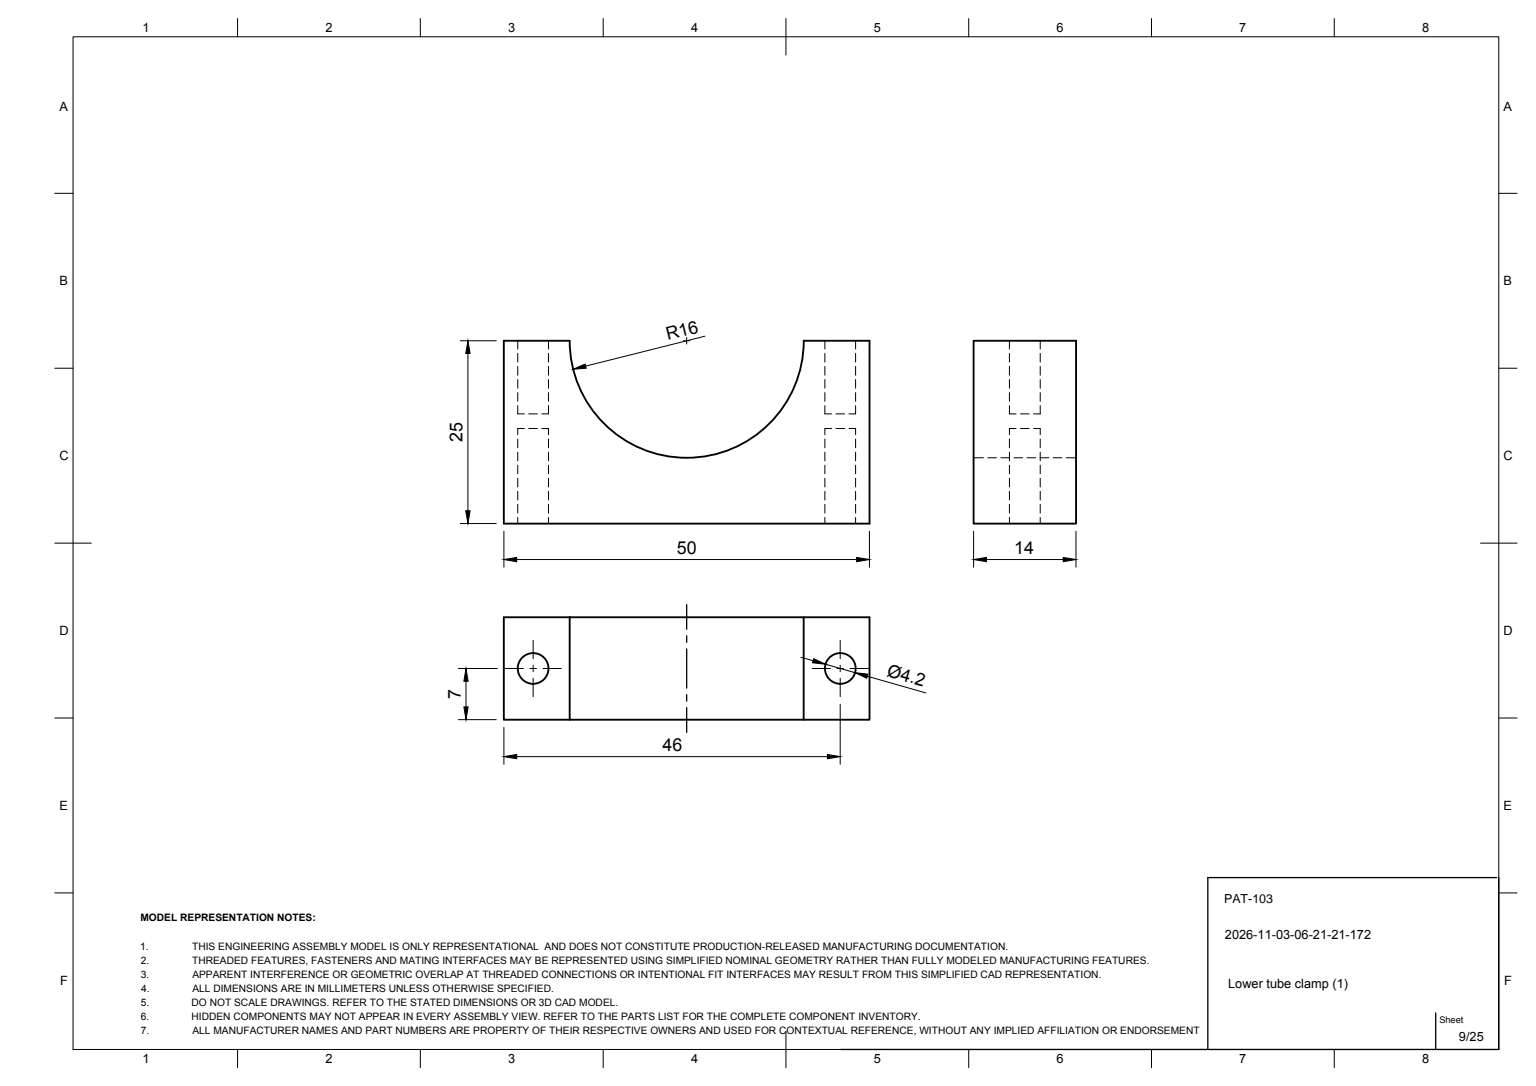
ISO-10303-21;
HEADER;
/* Generated by software containing ST-Developer
 * from STEP Tools, Inc. (www.steptools.com) 
 */

FILE_DESCRIPTION(
/* description */ ('Telescoping shaft support with lock collar'),
/* implementation_level */ '2;1');

FILE_NAME(
/* name */ 'Lower tube clamp (1).step',
/* time_stamp */ '2026-10-27T10:48:51-07:00',
/* author */ (''),
/* organization */ (''),
/* preprocessor_version */ 'ST-DEVELOPER v20.2',
/* originating_system */ 'Autodesk Translation Framework v15.17.0.0',
/* authorisation */ '');

FILE_SCHEMA (('AUTOMOTIVE_DESIGN { 1 0 10303 214 3 1 1 }'));
ENDSEC;

DATA;
#10=MECHANICAL_DESIGN_GEOMETRIC_PRESENTATION_REPRESENTATION('',(#245),#7349);
#205=SHAPE_REPRESENTATION_RELATIONSHIP('SRR','None',#7447,#225);
#225=ADVANCED_BREP_SHAPE_REPRESENTATION('',(#265),#7331);
#245=STYLED_ITEM('',(#7613),#265);
#265=MANIFOLD_SOLID_BREP('Body1',#3968);
#305=FACE_BOUND('',#818,.T.);
#306=FACE_BOUND('',#823,.T.);
#307=FACE_BOUND('',#825,.T.);
#308=FACE_BOUND('',#826,.T.);
#395=PLANE('',#4349);
#396=PLANE('',#4353);
#397=PLANE('',#4357);
#398=PLANE('',#4361);
#399=PLANE('',#4365);
#400=PLANE('',#4366);
#401=PLANE('',#4367);
#402=PLANE('',#4368);
#403=PLANE('',#4369);
#404=PLANE('',#4370);
#405=PLANE('',#4371);
#555=FACE_OUTER_BOUND('',#807,.T.);
#556=FACE_OUTER_BOUND('',#808,.T.);
#557=FACE_OUTER_BOUND('',#809,.T.);
#558=FACE_OUTER_BOUND('',#810,.T.);
#559=FACE_OUTER_BOUND('',#811,.T.);
#560=FACE_OUTER_BOUND('',#812,.T.);
#561=FACE_OUTER_BOUND('',#813,.T.);
#562=FACE_OUTER_BOUND('',#814,.T.);
#563=FACE_OUTER_BOUND('',#815,.T.);
#564=FACE_OUTER_BOUND('',#816,.T.);
#565=FACE_OUTER_BOUND('',#817,.T.);
#566=FACE_OUTER_BOUND('',#819,.T.);
#567=FACE_OUTER_BOUND('',#820,.T.);
#568=FACE_OUTER_BOUND('',#821,.T.);
#569=FACE_OUTER_BOUND('',#822,.T.);
#570=FACE_OUTER_BOUND('',#824,.T.);
#807=EDGE_LOOP('',(#2954,#2955,#2956,#2957));
#808=EDGE_LOOP('',(#2958));
#809=EDGE_LOOP('',(#2959,#2960,#2961,#2962));
#810=EDGE_LOOP('',(#2963));
#811=EDGE_LOOP('',(#2964,#2965,#2966,#2967));
#812=EDGE_LOOP('',(#2968));
#813=EDGE_LOOP('',(#2969,#2970,#2971,#2972));
#814=EDGE_LOOP('',(#2973));
#815=EDGE_LOOP('',(#2974,#2975,#2976,#2977));
#816=EDGE_LOOP('',(#2978,#2979,#2980,#2981,#2982,#2983));
#817=EDGE_LOOP('',(#2984,#2985,#2986,#2987));
#818=EDGE_LOOP('',(#2988));
#819=EDGE_LOOP('',(#2989,#2990,#2991,#2992));
#820=EDGE_LOOP('',(#2993,#2994,#2995,#2996));
#821=EDGE_LOOP('',(#2997,#2998,#2999,#3000,#3001,#3002));
#822=EDGE_LOOP('',(#3003,#3004,#3005,#3006));
#823=EDGE_LOOP('',(#3007));
#824=EDGE_LOOP('',(#3008,#3009,#3010,#3011));
#825=EDGE_LOOP('',(#3012));
#826=EDGE_LOOP('',(#3013));
#1111=LINE('',#6318,#1391);
#1112=LINE('',#6325,#1392);
#1113=LINE('',#6332,#1393);
#1114=LINE('',#6339,#1394);
#1115=LINE('',#6347,#1395);
#1116=LINE('',#6350,#1396);
#1117=LINE('',#6353,#1397);
#1118=LINE('',#6355,#1398);
#1119=LINE('',#6357,#1399);
#1120=LINE('',#6359,#1400);
#1121=LINE('',#6360,#1401);
#1122=LINE('',#6363,#1402);
#1123=LINE('',#6364,#1403);
#1124=LINE('',#6367,#1404);
#1125=LINE('',#6369,#1405);
#1126=LINE('',#6370,#1406);
#1127=LINE('',#6373,#1407);
#1128=LINE('',#6374,#1408);
#1129=LINE('',#6376,#1409);
#1130=LINE('',#6377,#1410);
#1391=VECTOR('',#5073,0.21);
#1392=VECTOR('',#5082,0.21);
#1393=VECTOR('',#5091,0.21);
#1394=VECTOR('',#5100,0.21);
#1395=VECTOR('',#5109,1.);
#1396=VECTOR('',#5112,1.);
#1397=VECTOR('',#5115,1.);
#1398=VECTOR('',#5116,1.);
#1399=VECTOR('',#5117,1.);
#1400=VECTOR('',#5118,1.);
#1401=VECTOR('',#5119,1.);
#1402=VECTOR('',#5122,1.);
#1403=VECTOR('',#5123,1.);
#1404=VECTOR('',#5126,1.);
#1405=VECTOR('',#5127,1.);
#1406=VECTOR('',#5128,1.);
#1407=VECTOR('',#5131,1.);
#1408=VECTOR('',#5132,1.);
#1409=VECTOR('',#5135,1.);
#1410=VECTOR('',#5136,1.);
#1659=CIRCLE('',#4347,0.21);
#1660=CIRCLE('',#4348,0.21);
#1661=CIRCLE('',#4351,0.21);
#1662=CIRCLE('',#4352,0.21);
#1663=CIRCLE('',#4355,0.21);
#1664=CIRCLE('',#4356,0.21);
#1665=CIRCLE('',#4359,0.21);
#1666=CIRCLE('',#4360,0.21);
#1667=CIRCLE('',#4363,1.6);
#1668=CIRCLE('',#4364,1.6);
#1902=VERTEX_POINT('',#6315);
#1903=VERTEX_POINT('',#6317);
#1904=VERTEX_POINT('',#6322);
#1905=VERTEX_POINT('',#6324);
#1906=VERTEX_POINT('',#6329);
#1907=VERTEX_POINT('',#6331);
#1908=VERTEX_POINT('',#6336);
#1909=VERTEX_POINT('',#6338);
#1910=VERTEX_POINT('',#6343);
#1911=VERTEX_POINT('',#6344);
#1912=VERTEX_POINT('',#6346);
#1913=VERTEX_POINT('',#6348);
#1914=VERTEX_POINT('',#6352);
#1915=VERTEX_POINT('',#6354);
#1916=VERTEX_POINT('',#6356);
#1917=VERTEX_POINT('',#6358);
#1918=VERTEX_POINT('',#6362);
#1919=VERTEX_POINT('',#6366);
#1920=VERTEX_POINT('',#6368);
#1921=VERTEX_POINT('',#6372);
#2289=EDGE_CURVE('',#1902,#1902,#1659,.T.);
#2290=EDGE_CURVE('',#1902,#1903,#1111,.T.);
#2291=EDGE_CURVE('',#1903,#1903,#1660,.T.);
#2292=EDGE_CURVE('',#1904,#1904,#1661,.T.);
#2293=EDGE_CURVE('',#1904,#1905,#1112,.T.);
#2294=EDGE_CURVE('',#1905,#1905,#1662,.T.);
#2295=EDGE_CURVE('',#1906,#1906,#1663,.T.);
#2296=EDGE_CURVE('',#1906,#1907,#1113,.T.);
#2297=EDGE_CURVE('',#1907,#1907,#1664,.T.);
#2298=EDGE_CURVE('',#1908,#1908,#1665,.T.);
#2299=EDGE_CURVE('',#1908,#1909,#1114,.T.);
#2300=EDGE_CURVE('',#1909,#1909,#1666,.T.);
#2301=EDGE_CURVE('',#1910,#1911,#1667,.T.);
#2302=EDGE_CURVE('',#1912,#1910,#1115,.T.);
#2303=EDGE_CURVE('',#1913,#1912,#1668,.T.);
#2304=EDGE_CURVE('',#1911,#1913,#1116,.T.);
#2305=EDGE_CURVE('',#1914,#1912,#1117,.T.);
#2306=EDGE_CURVE('',#1915,#1914,#1118,.T.);
#2307=EDGE_CURVE('',#1915,#1916,#1119,.T.);
#2308=EDGE_CURVE('',#1916,#1917,#1120,.T.);
#2309=EDGE_CURVE('',#1913,#1917,#1121,.T.);
#2310=EDGE_CURVE('',#1910,#1918,#1122,.T.);
#2311=EDGE_CURVE('',#1918,#1914,#1123,.T.);
#2312=EDGE_CURVE('',#1916,#1919,#1124,.T.);
#2313=EDGE_CURVE('',#1919,#1920,#1125,.T.);
#2314=EDGE_CURVE('',#1917,#1920,#1126,.T.);
#2315=EDGE_CURVE('',#1921,#1915,#1127,.T.);
#2316=EDGE_CURVE('',#1921,#1918,#1128,.T.);
#2317=EDGE_CURVE('',#1920,#1911,#1129,.T.);
#2318=EDGE_CURVE('',#1919,#1921,#1130,.T.);
#2954=ORIENTED_EDGE('',*,*,#2289,.F.);
#2955=ORIENTED_EDGE('',*,*,#2290,.T.);
#2956=ORIENTED_EDGE('',*,*,#2291,.F.);
#2957=ORIENTED_EDGE('',*,*,#2290,.F.);
#2958=ORIENTED_EDGE('',*,*,#2289,.T.);
#2959=ORIENTED_EDGE('',*,*,#2292,.F.);
#2960=ORIENTED_EDGE('',*,*,#2293,.T.);
#2961=ORIENTED_EDGE('',*,*,#2294,.F.);
#2962=ORIENTED_EDGE('',*,*,#2293,.F.);
#2963=ORIENTED_EDGE('',*,*,#2292,.T.);
#2964=ORIENTED_EDGE('',*,*,#2295,.F.);
#2965=ORIENTED_EDGE('',*,*,#2296,.T.);
#2966=ORIENTED_EDGE('',*,*,#2297,.T.);
#2967=ORIENTED_EDGE('',*,*,#2296,.F.);
#2968=ORIENTED_EDGE('',*,*,#2297,.F.);
#2969=ORIENTED_EDGE('',*,*,#2298,.F.);
#2970=ORIENTED_EDGE('',*,*,#2299,.T.);
#2971=ORIENTED_EDGE('',*,*,#2300,.T.);
#2972=ORIENTED_EDGE('',*,*,#2299,.F.);
#2973=ORIENTED_EDGE('',*,*,#2300,.F.);
#2974=ORIENTED_EDGE('',*,*,#2301,.F.);
#2975=ORIENTED_EDGE('',*,*,#2302,.F.);
#2976=ORIENTED_EDGE('',*,*,#2303,.F.);
#2977=ORIENTED_EDGE('',*,*,#2304,.F.);
#2978=ORIENTED_EDGE('',*,*,#2303,.T.);
#2979=ORIENTED_EDGE('',*,*,#2305,.F.);
#2980=ORIENTED_EDGE('',*,*,#2306,.F.);
#2981=ORIENTED_EDGE('',*,*,#2307,.T.);
#2982=ORIENTED_EDGE('',*,*,#2308,.T.);
#2983=ORIENTED_EDGE('',*,*,#2309,.F.);
#2984=ORIENTED_EDGE('',*,*,#2302,.T.);
#2985=ORIENTED_EDGE('',*,*,#2310,.T.);
#2986=ORIENTED_EDGE('',*,*,#2311,.T.);
#2987=ORIENTED_EDGE('',*,*,#2305,.T.);
#2988=ORIENTED_EDGE('',*,*,#2291,.T.);
#2989=ORIENTED_EDGE('',*,*,#2312,.T.);
#2990=ORIENTED_EDGE('',*,*,#2313,.T.);
#2991=ORIENTED_EDGE('',*,*,#2314,.F.);
#2992=ORIENTED_EDGE('',*,*,#2308,.F.);
#2993=ORIENTED_EDGE('',*,*,#2315,.T.);
#2994=ORIENTED_EDGE('',*,*,#2306,.T.);
#2995=ORIENTED_EDGE('',*,*,#2311,.F.);
#2996=ORIENTED_EDGE('',*,*,#2316,.F.);
#2997=ORIENTED_EDGE('',*,*,#2301,.T.);
#2998=ORIENTED_EDGE('',*,*,#2317,.F.);
#2999=ORIENTED_EDGE('',*,*,#2313,.F.);
#3000=ORIENTED_EDGE('',*,*,#2318,.T.);
#3001=ORIENTED_EDGE('',*,*,#2316,.T.);
#3002=ORIENTED_EDGE('',*,*,#2310,.F.);
#3003=ORIENTED_EDGE('',*,*,#2304,.T.);
#3004=ORIENTED_EDGE('',*,*,#2309,.T.);
#3005=ORIENTED_EDGE('',*,*,#2314,.T.);
#3006=ORIENTED_EDGE('',*,*,#2317,.T.);
#3007=ORIENTED_EDGE('',*,*,#2294,.T.);
#3008=ORIENTED_EDGE('',*,*,#2318,.F.);
#3009=ORIENTED_EDGE('',*,*,#2312,.F.);
#3010=ORIENTED_EDGE('',*,*,#2307,.F.);
#3011=ORIENTED_EDGE('',*,*,#2315,.F.);
#3012=ORIENTED_EDGE('',*,*,#2295,.T.);
#3013=ORIENTED_EDGE('',*,*,#2298,.T.);
#3684=CYLINDRICAL_SURFACE('',#4346,0.21);
#3685=CYLINDRICAL_SURFACE('',#4350,0.21);
#3686=CYLINDRICAL_SURFACE('',#4354,0.21);
#3687=CYLINDRICAL_SURFACE('',#4358,0.21);
#3688=CYLINDRICAL_SURFACE('',#4362,1.6);
#3798=ADVANCED_FACE('',(#555),#3684,.F.);
#3799=ADVANCED_FACE('',(#556),#395,.T.);
#3800=ADVANCED_FACE('',(#557),#3685,.F.);
#3801=ADVANCED_FACE('',(#558),#396,.T.);
#3802=ADVANCED_FACE('',(#559),#3686,.F.);
#3803=ADVANCED_FACE('',(#560),#397,.F.);
#3804=ADVANCED_FACE('',(#561),#3687,.F.);
#3805=ADVANCED_FACE('',(#562),#398,.F.);
#3806=ADVANCED_FACE('',(#563),#3688,.F.);
#3807=ADVANCED_FACE('',(#564),#399,.T.);
#3808=ADVANCED_FACE('',(#565,#305),#400,.T.);
#3809=ADVANCED_FACE('',(#566),#401,.T.);
#3810=ADVANCED_FACE('',(#567),#402,.T.);
#3811=ADVANCED_FACE('',(#568),#403,.T.);
#3812=ADVANCED_FACE('',(#569,#306),#404,.T.);
#3813=ADVANCED_FACE('',(#570,#307,#308),#405,.F.);
#3968=CLOSED_SHELL('',(#3798,#3799,#3800,#3801,#3802,#3803,#3804,#3805,
#3806,#3807,#3808,#3809,#3810,#3811,#3812,#3813));
#4345=AXIS2_PLACEMENT_3D('',#6313,#5067,#5068);
#4346=AXIS2_PLACEMENT_3D('',#6314,#5069,#5070);
#4347=AXIS2_PLACEMENT_3D('',#6316,#5071,#5072);
#4348=AXIS2_PLACEMENT_3D('',#6319,#5074,#5075);
#4349=AXIS2_PLACEMENT_3D('',#6320,#5076,#5077);
#4350=AXIS2_PLACEMENT_3D('',#6321,#5078,#5079);
#4351=AXIS2_PLACEMENT_3D('',#6323,#5080,#5081);
#4352=AXIS2_PLACEMENT_3D('',#6326,#5083,#5084);
#4353=AXIS2_PLACEMENT_3D('',#6327,#5085,#5086);
#4354=AXIS2_PLACEMENT_3D('',#6328,#5087,#5088);
#4355=AXIS2_PLACEMENT_3D('',#6330,#5089,#5090);
#4356=AXIS2_PLACEMENT_3D('',#6333,#5092,#5093);
#4357=AXIS2_PLACEMENT_3D('',#6334,#5094,#5095);
#4358=AXIS2_PLACEMENT_3D('',#6335,#5096,#5097);
#4359=AXIS2_PLACEMENT_3D('',#6337,#5098,#5099);
#4360=AXIS2_PLACEMENT_3D('',#6340,#5101,#5102);
#4361=AXIS2_PLACEMENT_3D('',#6341,#5103,#5104);
#4362=AXIS2_PLACEMENT_3D('',#6342,#5105,#5106);
#4363=AXIS2_PLACEMENT_3D('',#6345,#5107,#5108);
#4364=AXIS2_PLACEMENT_3D('',#6349,#5110,#5111);
#4365=AXIS2_PLACEMENT_3D('',#6351,#5113,#5114);
#4366=AXIS2_PLACEMENT_3D('',#6361,#5120,#5121);
#4367=AXIS2_PLACEMENT_3D('',#6365,#5124,#5125);
#4368=AXIS2_PLACEMENT_3D('',#6371,#5129,#5130);
#4369=AXIS2_PLACEMENT_3D('',#6375,#5133,#5134);
#4370=AXIS2_PLACEMENT_3D('',#6378,#5137,#5138);
#4371=AXIS2_PLACEMENT_3D('',#6379,#5139,#5140);
#5067=DIRECTION('axis',(0.,0.,1.));
#5068=DIRECTION('refdir',(1.,0.,0.));
#5069=DIRECTION('center_axis',(0.,0.,1.));
#5070=DIRECTION('ref_axis',(1.,0.,0.));
#5071=DIRECTION('center_axis',(0.,0.,1.));
#5072=DIRECTION('ref_axis',(1.,0.,0.));
#5073=DIRECTION('',(0.,0.,1.));
#5074=DIRECTION('center_axis',(0.,0.,-1.));
#5075=DIRECTION('ref_axis',(1.,0.,0.));
#5076=DIRECTION('center_axis',(0.,0.,1.));
#5077=DIRECTION('ref_axis',(1.,0.,0.));
#5078=DIRECTION('center_axis',(0.,0.,1.));
#5079=DIRECTION('ref_axis',(1.,0.,0.));
#5080=DIRECTION('center_axis',(0.,0.,1.));
#5081=DIRECTION('ref_axis',(1.,0.,0.));
#5082=DIRECTION('',(0.,0.,1.));
#5083=DIRECTION('center_axis',(0.,0.,-1.));
#5084=DIRECTION('ref_axis',(1.,0.,0.));
#5085=DIRECTION('center_axis',(0.,0.,1.));
#5086=DIRECTION('ref_axis',(1.,0.,0.));
#5087=DIRECTION('center_axis',(0.,0.,1.));
#5088=DIRECTION('ref_axis',(1.,0.,0.));
#5089=DIRECTION('center_axis',(0.,0.,1.));
#5090=DIRECTION('ref_axis',(1.,0.,0.));
#5091=DIRECTION('',(0.,0.,1.));
#5092=DIRECTION('center_axis',(0.,0.,1.));
#5093=DIRECTION('ref_axis',(1.,0.,0.));
#5094=DIRECTION('center_axis',(0.,0.,1.));
#5095=DIRECTION('ref_axis',(1.,0.,0.));
#5096=DIRECTION('center_axis',(0.,0.,1.));
#5097=DIRECTION('ref_axis',(1.,0.,0.));
#5098=DIRECTION('center_axis',(0.,0.,1.));
#5099=DIRECTION('ref_axis',(1.,0.,0.));
#5100=DIRECTION('',(0.,0.,1.));
#5101=DIRECTION('center_axis',(0.,0.,1.));
#5102=DIRECTION('ref_axis',(1.,0.,0.));
#5103=DIRECTION('center_axis',(0.,0.,1.));
#5104=DIRECTION('ref_axis',(1.,0.,0.));
#5105=DIRECTION('center_axis',(1.,0.,0.));
#5106=DIRECTION('ref_axis',(0.,0.,-1.));
#5107=DIRECTION('center_axis',(1.,0.,0.));
#5108=DIRECTION('ref_axis',(0.,0.,-1.));
#5109=DIRECTION('',(-1.,0.,0.));
#5110=DIRECTION('center_axis',(-1.,0.,0.));
#5111=DIRECTION('ref_axis',(0.,0.,-1.));
#5112=DIRECTION('',(1.,0.,0.));
#5113=DIRECTION('center_axis',(1.,0.,0.));
#5114=DIRECTION('ref_axis',(0.,1.,0.));
#5115=DIRECTION('',(0.,1.,0.));
#5116=DIRECTION('',(0.,0.,1.));
#5117=DIRECTION('',(0.,1.,0.));
#5118=DIRECTION('',(0.,0.,1.));
#5119=DIRECTION('',(0.,1.,0.));
#5120=DIRECTION('center_axis',(0.,0.,1.));
#5121=DIRECTION('ref_axis',(1.,0.,0.));
#5122=DIRECTION('',(0.,-1.,0.));
#5123=DIRECTION('',(1.,0.,0.));
#5124=DIRECTION('center_axis',(0.,1.,0.));
#5125=DIRECTION('ref_axis',(-1.,0.,0.));
#5126=DIRECTION('',(-1.,0.,0.));
#5127=DIRECTION('',(0.,0.,1.));
#5128=DIRECTION('',(-1.,0.,0.));
#5129=DIRECTION('center_axis',(0.,-1.,0.));
#5130=DIRECTION('ref_axis',(1.,0.,0.));
#5131=DIRECTION('',(1.,0.,0.));
#5132=DIRECTION('',(0.,0.,1.));
#5133=DIRECTION('center_axis',(-1.,0.,0.));
#5134=DIRECTION('ref_axis',(0.,-1.,0.));
#5135=DIRECTION('',(0.,-1.,0.));
#5136=DIRECTION('',(0.,-1.,0.));
#5137=DIRECTION('center_axis',(0.,0.,1.));
#5138=DIRECTION('ref_axis',(1.,0.,0.));
#5139=DIRECTION('center_axis',(0.,0.,1.));
#5140=DIRECTION('ref_axis',(1.,0.,0.));
#6313=CARTESIAN_POINT('',(0.,0.,0.));
#6314=CARTESIAN_POINT('Origin',(7.8,-2.1,2.5));
#6315=CARTESIAN_POINT('',(7.59,-2.1,2.5));
#6316=CARTESIAN_POINT('Origin',(7.8,-2.1,2.5));
#6317=CARTESIAN_POINT('',(7.59,-2.1,3.5));
#6318=CARTESIAN_POINT('',(7.59,-2.1,2.5));
#6319=CARTESIAN_POINT('Origin',(7.8,-2.1,3.5));
#6320=CARTESIAN_POINT('Origin',(7.8,-2.1,2.5));
#6321=CARTESIAN_POINT('Origin',(7.8,2.1,2.5));
#6322=CARTESIAN_POINT('',(7.59,2.1,2.5));
#6323=CARTESIAN_POINT('Origin',(7.8,2.1,2.5));
#6324=CARTESIAN_POINT('',(7.59,2.1,3.5));
#6325=CARTESIAN_POINT('',(7.59,2.1,2.5));
#6326=CARTESIAN_POINT('Origin',(7.8,2.1,3.5));
#6327=CARTESIAN_POINT('Origin',(7.8,2.1,2.5));
#6328=CARTESIAN_POINT('Origin',(7.8,-2.1,0.9));
#6329=CARTESIAN_POINT('',(7.59,-2.1,1.));
#6330=CARTESIAN_POINT('Origin',(7.8,-2.1,1.));
#6331=CARTESIAN_POINT('',(7.59,-2.1,2.3));
#6332=CARTESIAN_POINT('',(7.59,-2.1,0.9));
#6333=CARTESIAN_POINT('Origin',(7.8,-2.1,2.3));
#6334=CARTESIAN_POINT('Origin',(7.8,-2.1,2.3));
#6335=CARTESIAN_POINT('Origin',(7.8,2.1,0.9));
#6336=CARTESIAN_POINT('',(7.59,2.1,1.));
#6337=CARTESIAN_POINT('Origin',(7.8,2.1,1.));
#6338=CARTESIAN_POINT('',(7.59,2.1,2.3));
#6339=CARTESIAN_POINT('',(7.59,2.1,0.9));
#6340=CARTESIAN_POINT('Origin',(7.8,2.1,2.3));
#6341=CARTESIAN_POINT('Origin',(7.8,2.1,2.3));
#6342=CARTESIAN_POINT('Origin',(7.,0.,3.5));
#6343=CARTESIAN_POINT('',(7.1,-1.6,3.5));
#6344=CARTESIAN_POINT('',(7.1,1.6,3.5));
#6345=CARTESIAN_POINT('Origin',(7.1,0.,3.5));
#6346=CARTESIAN_POINT('',(8.5,-1.6,3.5));
#6347=CARTESIAN_POINT('',(7.,-1.6,3.5));
#6348=CARTESIAN_POINT('',(8.5,1.6,3.5));
#6349=CARTESIAN_POINT('Origin',(8.5,0.,3.5));
#6350=CARTESIAN_POINT('',(7.,1.6,3.5));
#6351=CARTESIAN_POINT('Origin',(8.5,-2.5,1.));
#6352=CARTESIAN_POINT('',(8.5,-2.5,3.5));
#6353=CARTESIAN_POINT('',(8.5,-2.5,3.5));
#6354=CARTESIAN_POINT('',(8.5,-2.5,1.));
#6355=CARTESIAN_POINT('',(8.5,-2.5,1.));
#6356=CARTESIAN_POINT('',(8.5,2.5,1.));
#6357=CARTESIAN_POINT('',(8.5,-2.5,1.));
#6358=CARTESIAN_POINT('',(8.5,2.5,3.5));
#6359=CARTESIAN_POINT('',(8.5,2.5,1.));
#6360=CARTESIAN_POINT('',(8.5,-2.5,3.5));
#6361=CARTESIAN_POINT('Origin',(7.8,0.,3.5));
#6362=CARTESIAN_POINT('',(7.1,-2.5,3.5));
#6363=CARTESIAN_POINT('',(7.1,2.5,3.5));
#6364=CARTESIAN_POINT('',(7.1,-2.5,3.5));
#6365=CARTESIAN_POINT('Origin',(8.5,2.5,1.));
#6366=CARTESIAN_POINT('',(7.1,2.5,1.));
#6367=CARTESIAN_POINT('',(8.5,2.5,1.));
#6368=CARTESIAN_POINT('',(7.1,2.5,3.5));
#6369=CARTESIAN_POINT('',(7.1,2.5,1.));
#6370=CARTESIAN_POINT('',(8.5,2.5,3.5));
#6371=CARTESIAN_POINT('Origin',(7.1,-2.5,1.));
#6372=CARTESIAN_POINT('',(7.1,-2.5,1.));
#6373=CARTESIAN_POINT('',(7.1,-2.5,1.));
#6374=CARTESIAN_POINT('',(7.1,-2.5,1.));
#6375=CARTESIAN_POINT('Origin',(7.1,2.5,1.));
#6376=CARTESIAN_POINT('',(7.1,2.5,3.5));
#6377=CARTESIAN_POINT('',(7.1,2.5,1.));
#6378=CARTESIAN_POINT('Origin',(7.8,0.,3.5));
#6379=CARTESIAN_POINT('Origin',(7.8,0.,1.));
#7306=UNCERTAINTY_MEASURE_WITH_UNIT(LENGTH_MEASURE(0.001),#7350,
'DISTANCE_ACCURACY_VALUE',
'Maximum model space distance between geometric entities at asserted c
onnectivities');
#7324=UNCERTAINTY_MEASURE_WITH_UNIT(LENGTH_MEASURE(0.001),#7350,
'DISTANCE_ACCURACY_VALUE',
'Maximum model space distance between geometric entities at asserted c
onnectivities');
#7331=(
GEOMETRIC_REPRESENTATION_CONTEXT(3)
GLOBAL_UNCERTAINTY_ASSIGNED_CONTEXT((#7306))
GLOBAL_UNIT_ASSIGNED_CONTEXT((#7350,#7352,#7353))
REPRESENTATION_CONTEXT('','3D')
);
#7349=(
GEOMETRIC_REPRESENTATION_CONTEXT(3)
GLOBAL_UNCERTAINTY_ASSIGNED_CONTEXT((#7324))
GLOBAL_UNIT_ASSIGNED_CONTEXT((#7350,#7352,#7353))
REPRESENTATION_CONTEXT('','3D')
);
#7350=(
LENGTH_UNIT()
NAMED_UNIT(*)
SI_UNIT(.CENTI.,.METRE.)
);
#7352=(
NAMED_UNIT(*)
PLANE_ANGLE_UNIT()
SI_UNIT($,.RADIAN.)
);
#7353=(
NAMED_UNIT(*)
SI_UNIT($,.STERADIAN.)
SOLID_ANGLE_UNIT()
);
#7360=SHAPE_DEFINITION_REPRESENTATION(#7384,#7447);
#7384=PRODUCT_DEFINITION_SHAPE('',$,#7472);
#7447=SHAPE_REPRESENTATION('',(#4345),#7331);
#7465=PRODUCT_DEFINITION_CONTEXT('part definition',#7539,'design');
#7472=PRODUCT_DEFINITION('Lower tube clamp (1)','Lower tube clamp (1)',#7496,
#7465);
#7496=PRODUCT_DEFINITION_FORMATION('',$,#7547);
#7539=APPLICATION_CONTEXT(
'Core Data for Automotive Mechanical Design Process');
#7540=PRODUCT_CONTEXT('part definition',#7539,'mechanical');
#7547=PRODUCT('Lower tube clamp (1)','Lower tube clamp (1)',
'Lower tube clamp (1)',(#7540));
#7607=COLOUR_RGB('Light Blue',0.38,0.62,0.78);
#7608=FILL_AREA_STYLE_COLOUR('',#7607);
#7609=FILL_AREA_STYLE('',(#7608));
#7610=SURFACE_STYLE_FILL_AREA(#7609);
#7611=SURFACE_SIDE_STYLE('',(#7610));
#7612=SURFACE_STYLE_USAGE(.BOTH.,#7611);
#7613=PRESENTATION_STYLE_ASSIGNMENT((#7612));
ENDSEC;
END-ISO-10303-21;
